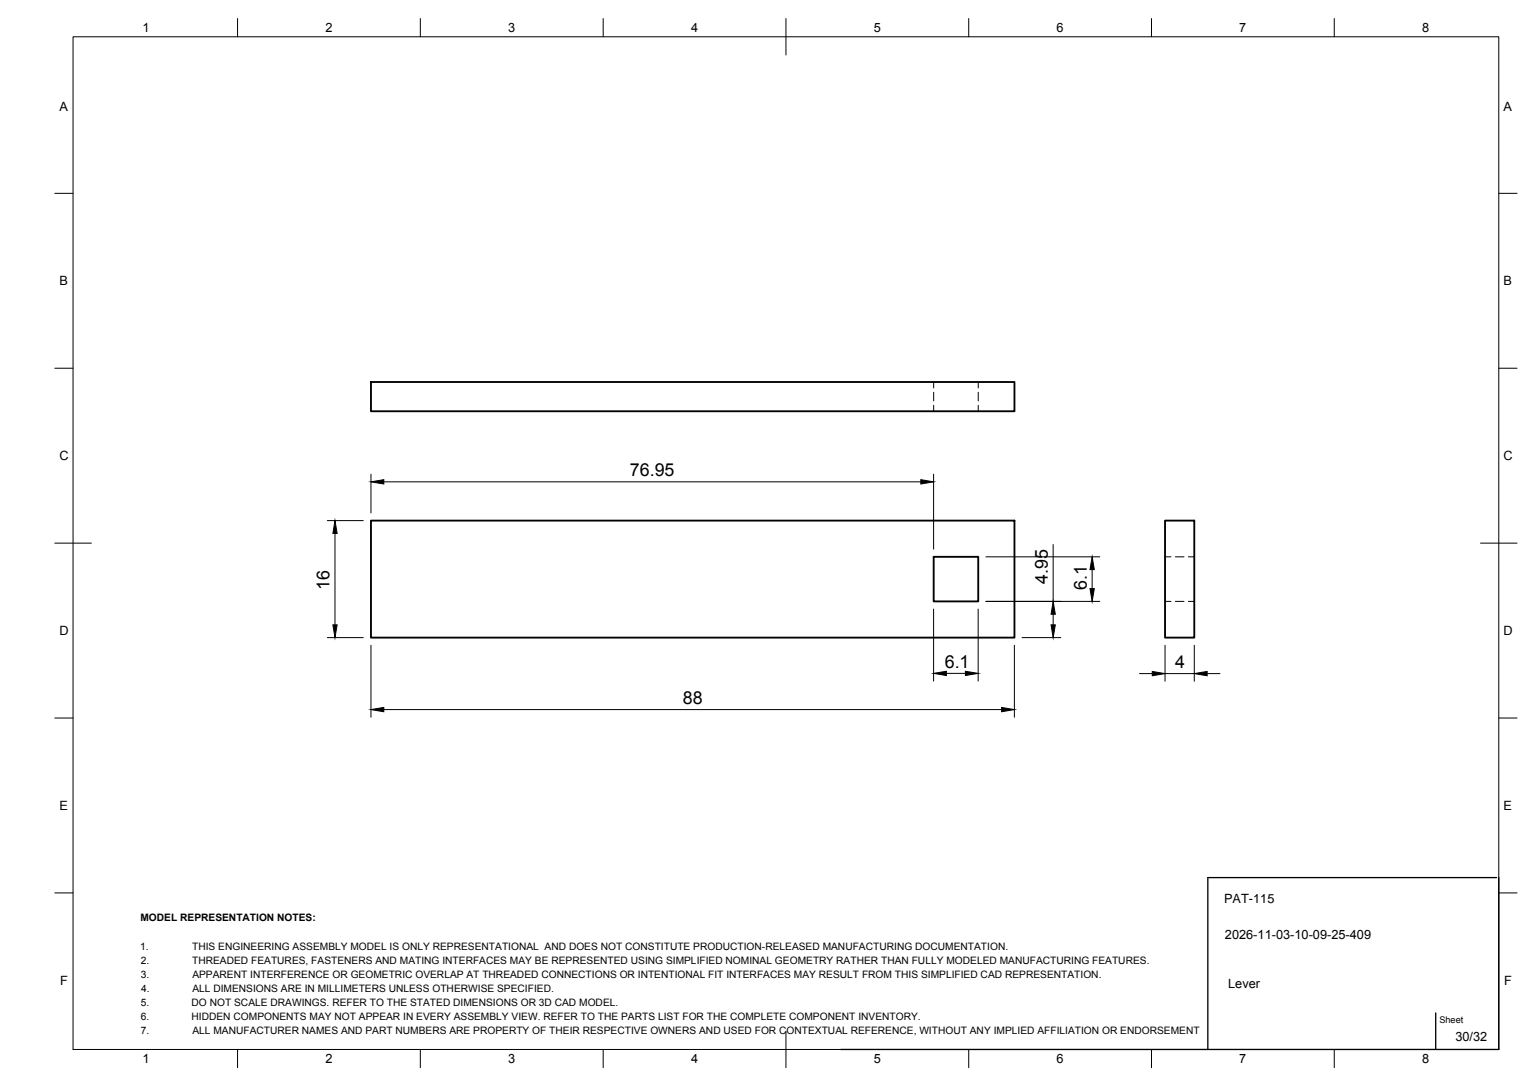
ISO-10303-21;
HEADER;
/* Generated by software containing ST-Developer
 * from STEP Tools, Inc. (www.steptools.com) 
 */

FILE_DESCRIPTION(
/* description */ ('Union bypass pipe loop'),
/* implementation_level */ '2;1');

FILE_NAME(
/* name */ 'Lever.step',
/* time_stamp */ '2026-10-27T21:00:29-07:00',
/* author */ (''),
/* organization */ (''),
/* preprocessor_version */ 'ST-DEVELOPER v20.2',
/* originating_system */ 'Autodesk Translation Framework v15.17.0.0',
/* authorisation */ '');

FILE_SCHEMA (('AUTOMOTIVE_DESIGN { 1 0 10303 214 3 1 1 }'));
ENDSEC;

DATA;
#10=MECHANICAL_DESIGN_GEOMETRIC_PRESENTATION_REPRESENTATION('',(#473),#10095);
#409=SHAPE_REPRESENTATION_RELATIONSHIP('SRR','None',#10279,#441);
#441=ADVANCED_BREP_SHAPE_REPRESENTATION('',(#502),#10091);
#473=STYLED_ITEM('',(#10514),#502);
#502=MANIFOLD_SOLID_BREP('Body1',#5547);
#630=FACE_BOUND('',#1591,.T.);
#631=FACE_BOUND('',#1593,.T.);
#806=PLANE('',#6561);
#807=PLANE('',#6562);
#808=PLANE('',#6563);
#809=PLANE('',#6564);
#810=PLANE('',#6565);
#811=PLANE('',#6566);
#812=PLANE('',#6567);
#813=PLANE('',#6568);
#814=PLANE('',#6569);
#815=PLANE('',#6570);
#1131=FACE_OUTER_BOUND('',#1582,.T.);
#1132=FACE_OUTER_BOUND('',#1583,.T.);
#1133=FACE_OUTER_BOUND('',#1584,.T.);
#1134=FACE_OUTER_BOUND('',#1585,.T.);
#1135=FACE_OUTER_BOUND('',#1586,.T.);
#1136=FACE_OUTER_BOUND('',#1587,.T.);
#1137=FACE_OUTER_BOUND('',#1588,.T.);
#1138=FACE_OUTER_BOUND('',#1589,.T.);
#1139=FACE_OUTER_BOUND('',#1590,.T.);
#1140=FACE_OUTER_BOUND('',#1592,.T.);
#1582=EDGE_LOOP('',(#4936,#4937,#4938,#4939));
#1583=EDGE_LOOP('',(#4940,#4941,#4942,#4943));
#1584=EDGE_LOOP('',(#4944,#4945,#4946,#4947));
#1585=EDGE_LOOP('',(#4948,#4949,#4950,#4951));
#1586=EDGE_LOOP('',(#4952,#4953,#4954,#4955));
#1587=EDGE_LOOP('',(#4956,#4957,#4958,#4959));
#1588=EDGE_LOOP('',(#4960,#4961,#4962,#4963));
#1589=EDGE_LOOP('',(#4964,#4965,#4966,#4967));
#1590=EDGE_LOOP('',(#4968,#4969,#4970,#4971));
#1591=EDGE_LOOP('',(#4972,#4973,#4974,#4975));
#1592=EDGE_LOOP('',(#4976,#4977,#4978,#4979));
#1593=EDGE_LOOP('',(#4980,#4981,#4982,#4983));
#1938=LINE('',#9859,#2314);
#1939=LINE('',#9861,#2315);
#1940=LINE('',#9863,#2316);
#1941=LINE('',#9864,#2317);
#1942=LINE('',#9867,#2318);
#1943=LINE('',#9869,#2319);
#1944=LINE('',#9870,#2320);
#1945=LINE('',#9873,#2321);
#1946=LINE('',#9875,#2322);
#1947=LINE('',#9876,#2323);
#1948=LINE('',#9878,#2324);
#1949=LINE('',#9879,#2325);
#1950=LINE('',#9883,#2326);
#1951=LINE('',#9885,#2327);
#1952=LINE('',#9887,#2328);
#1953=LINE('',#9888,#2329);
#1954=LINE('',#9891,#2330);
#1955=LINE('',#9893,#2331);
#1956=LINE('',#9894,#2332);
#1957=LINE('',#9897,#2333);
#1958=LINE('',#9899,#2334);
#1959=LINE('',#9900,#2335);
#1960=LINE('',#9902,#2336);
#1961=LINE('',#9903,#2337);
#2314=VECTOR('',#8248,1.);
#2315=VECTOR('',#8249,1.);
#2316=VECTOR('',#8250,1.);
#2317=VECTOR('',#8251,1.);
#2318=VECTOR('',#8254,1.);
#2319=VECTOR('',#8255,1.);
#2320=VECTOR('',#8256,1.);
#2321=VECTOR('',#8259,1.);
#2322=VECTOR('',#8260,1.);
#2323=VECTOR('',#8261,1.);
#2324=VECTOR('',#8264,1.);
#2325=VECTOR('',#8265,1.);
#2326=VECTOR('',#8268,1.);
#2327=VECTOR('',#8269,1.);
#2328=VECTOR('',#8270,1.);
#2329=VECTOR('',#8271,1.);
#2330=VECTOR('',#8274,1.);
#2331=VECTOR('',#8275,1.);
#2332=VECTOR('',#8276,1.);
#2333=VECTOR('',#8279,1.);
#2334=VECTOR('',#8280,1.);
#2335=VECTOR('',#8281,1.);
#2336=VECTOR('',#8284,1.);
#2337=VECTOR('',#8285,1.);
#3020=VERTEX_POINT('',#9857);
#3021=VERTEX_POINT('',#9858);
#3022=VERTEX_POINT('',#9860);
#3023=VERTEX_POINT('',#9862);
#3024=VERTEX_POINT('',#9866);
#3025=VERTEX_POINT('',#9868);
#3026=VERTEX_POINT('',#9872);
#3027=VERTEX_POINT('',#9874);
#3028=VERTEX_POINT('',#9881);
#3029=VERTEX_POINT('',#9882);
#3030=VERTEX_POINT('',#9884);
#3031=VERTEX_POINT('',#9886);
#3032=VERTEX_POINT('',#9890);
#3033=VERTEX_POINT('',#9892);
#3034=VERTEX_POINT('',#9896);
#3035=VERTEX_POINT('',#9898);
#3666=EDGE_CURVE('',#3020,#3021,#1938,.T.);
#3667=EDGE_CURVE('',#3022,#3020,#1939,.T.);
#3668=EDGE_CURVE('',#3023,#3022,#1940,.T.);
#3669=EDGE_CURVE('',#3023,#3021,#1941,.T.);
#3670=EDGE_CURVE('',#3021,#3024,#1942,.T.);
#3671=EDGE_CURVE('',#3025,#3023,#1943,.T.);
#3672=EDGE_CURVE('',#3025,#3024,#1944,.T.);
#3673=EDGE_CURVE('',#3024,#3026,#1945,.T.);
#3674=EDGE_CURVE('',#3027,#3025,#1946,.T.);
#3675=EDGE_CURVE('',#3027,#3026,#1947,.T.);
#3676=EDGE_CURVE('',#3026,#3020,#1948,.T.);
#3677=EDGE_CURVE('',#3022,#3027,#1949,.T.);
#3678=EDGE_CURVE('',#3028,#3029,#1950,.T.);
#3679=EDGE_CURVE('',#3029,#3030,#1951,.T.);
#3680=EDGE_CURVE('',#3031,#3030,#1952,.T.);
#3681=EDGE_CURVE('',#3028,#3031,#1953,.T.);
#3682=EDGE_CURVE('',#3032,#3028,#1954,.T.);
#3683=EDGE_CURVE('',#3033,#3031,#1955,.T.);
#3684=EDGE_CURVE('',#3032,#3033,#1956,.T.);
#3685=EDGE_CURVE('',#3034,#3032,#1957,.T.);
#3686=EDGE_CURVE('',#3035,#3033,#1958,.T.);
#3687=EDGE_CURVE('',#3034,#3035,#1959,.T.);
#3688=EDGE_CURVE('',#3029,#3034,#1960,.T.);
#3689=EDGE_CURVE('',#3030,#3035,#1961,.T.);
#4936=ORIENTED_EDGE('',*,*,#3666,.F.);
#4937=ORIENTED_EDGE('',*,*,#3667,.F.);
#4938=ORIENTED_EDGE('',*,*,#3668,.F.);
#4939=ORIENTED_EDGE('',*,*,#3669,.T.);
#4940=ORIENTED_EDGE('',*,*,#3670,.F.);
#4941=ORIENTED_EDGE('',*,*,#3669,.F.);
#4942=ORIENTED_EDGE('',*,*,#3671,.F.);
#4943=ORIENTED_EDGE('',*,*,#3672,.T.);
#4944=ORIENTED_EDGE('',*,*,#3673,.F.);
#4945=ORIENTED_EDGE('',*,*,#3672,.F.);
#4946=ORIENTED_EDGE('',*,*,#3674,.F.);
#4947=ORIENTED_EDGE('',*,*,#3675,.T.);
#4948=ORIENTED_EDGE('',*,*,#3676,.F.);
#4949=ORIENTED_EDGE('',*,*,#3675,.F.);
#4950=ORIENTED_EDGE('',*,*,#3677,.F.);
#4951=ORIENTED_EDGE('',*,*,#3667,.T.);
#4952=ORIENTED_EDGE('',*,*,#3678,.T.);
#4953=ORIENTED_EDGE('',*,*,#3679,.T.);
#4954=ORIENTED_EDGE('',*,*,#3680,.F.);
#4955=ORIENTED_EDGE('',*,*,#3681,.F.);
#4956=ORIENTED_EDGE('',*,*,#3682,.T.);
#4957=ORIENTED_EDGE('',*,*,#3681,.T.);
#4958=ORIENTED_EDGE('',*,*,#3683,.F.);
#4959=ORIENTED_EDGE('',*,*,#3684,.F.);
#4960=ORIENTED_EDGE('',*,*,#3685,.T.);
#4961=ORIENTED_EDGE('',*,*,#3684,.T.);
#4962=ORIENTED_EDGE('',*,*,#3686,.F.);
#4963=ORIENTED_EDGE('',*,*,#3687,.F.);
#4964=ORIENTED_EDGE('',*,*,#3688,.T.);
#4965=ORIENTED_EDGE('',*,*,#3687,.T.);
#4966=ORIENTED_EDGE('',*,*,#3689,.F.);
#4967=ORIENTED_EDGE('',*,*,#3679,.F.);
#4968=ORIENTED_EDGE('',*,*,#3689,.T.);
#4969=ORIENTED_EDGE('',*,*,#3686,.T.);
#4970=ORIENTED_EDGE('',*,*,#3683,.T.);
#4971=ORIENTED_EDGE('',*,*,#3680,.T.);
#4972=ORIENTED_EDGE('',*,*,#3673,.T.);
#4973=ORIENTED_EDGE('',*,*,#3676,.T.);
#4974=ORIENTED_EDGE('',*,*,#3666,.T.);
#4975=ORIENTED_EDGE('',*,*,#3670,.T.);
#4976=ORIENTED_EDGE('',*,*,#3688,.F.);
#4977=ORIENTED_EDGE('',*,*,#3678,.F.);
#4978=ORIENTED_EDGE('',*,*,#3682,.F.);
#4979=ORIENTED_EDGE('',*,*,#3685,.F.);
#4980=ORIENTED_EDGE('',*,*,#3674,.T.);
#4981=ORIENTED_EDGE('',*,*,#3671,.T.);
#4982=ORIENTED_EDGE('',*,*,#3668,.T.);
#4983=ORIENTED_EDGE('',*,*,#3677,.T.);
#5480=ADVANCED_FACE('',(#1131),#806,.F.);
#5481=ADVANCED_FACE('',(#1132),#807,.F.);
#5482=ADVANCED_FACE('',(#1133),#808,.F.);
#5483=ADVANCED_FACE('',(#1134),#809,.F.);
#5484=ADVANCED_FACE('',(#1135),#810,.T.);
#5485=ADVANCED_FACE('',(#1136),#811,.T.);
#5486=ADVANCED_FACE('',(#1137),#812,.T.);
#5487=ADVANCED_FACE('',(#1138),#813,.T.);
#5488=ADVANCED_FACE('',(#1139,#630),#814,.T.);
#5489=ADVANCED_FACE('',(#1140,#631),#815,.F.);
#5547=CLOSED_SHELL('',(#5480,#5481,#5482,#5483,#5484,#5485,#5486,#5487,
#5488,#5489));
#6560=AXIS2_PLACEMENT_3D('',#9855,#8244,#8245);
#6561=AXIS2_PLACEMENT_3D('',#9856,#8246,#8247);
#6562=AXIS2_PLACEMENT_3D('',#9865,#8252,#8253);
#6563=AXIS2_PLACEMENT_3D('',#9871,#8257,#8258);
#6564=AXIS2_PLACEMENT_3D('',#9877,#8262,#8263);
#6565=AXIS2_PLACEMENT_3D('',#9880,#8266,#8267);
#6566=AXIS2_PLACEMENT_3D('',#9889,#8272,#8273);
#6567=AXIS2_PLACEMENT_3D('',#9895,#8277,#8278);
#6568=AXIS2_PLACEMENT_3D('',#9901,#8282,#8283);
#6569=AXIS2_PLACEMENT_3D('',#9904,#8286,#8287);
#6570=AXIS2_PLACEMENT_3D('',#9905,#8288,#8289);
#8244=DIRECTION('axis',(0.,0.,1.));
#8245=DIRECTION('refdir',(1.,0.,0.));
#8246=DIRECTION('center_axis',(0.,-1.,0.));
#8247=DIRECTION('ref_axis',(1.,0.,0.));
#8248=DIRECTION('',(-1.,0.,0.));
#8249=DIRECTION('',(0.,0.,1.));
#8250=DIRECTION('',(1.,0.,0.));
#8251=DIRECTION('',(0.,0.,1.));
#8252=DIRECTION('center_axis',(-1.,0.,0.));
#8253=DIRECTION('ref_axis',(0.,-1.,0.));
#8254=DIRECTION('',(0.,1.,0.));
#8255=DIRECTION('',(0.,-1.,0.));
#8256=DIRECTION('',(0.,0.,1.));
#8257=DIRECTION('center_axis',(0.,1.,0.));
#8258=DIRECTION('ref_axis',(-1.,0.,0.));
#8259=DIRECTION('',(1.,0.,0.));
#8260=DIRECTION('',(-1.,0.,0.));
#8261=DIRECTION('',(0.,0.,1.));
#8262=DIRECTION('center_axis',(1.,0.,0.));
#8263=DIRECTION('ref_axis',(0.,1.,0.));
#8264=DIRECTION('',(0.,-1.,0.));
#8265=DIRECTION('',(0.,1.,0.));
#8266=DIRECTION('center_axis',(0.,1.,0.));
#8267=DIRECTION('ref_axis',(-1.,0.,0.));
#8268=DIRECTION('',(-1.,0.,0.));
#8269=DIRECTION('',(0.,0.,1.));
#8270=DIRECTION('',(-1.,0.,0.));
#8271=DIRECTION('',(0.,0.,1.));
#8272=DIRECTION('center_axis',(1.,0.,0.));
#8273=DIRECTION('ref_axis',(0.,1.,0.));
#8274=DIRECTION('',(0.,1.,0.));
#8275=DIRECTION('',(0.,1.,0.));
#8276=DIRECTION('',(0.,0.,1.));
#8277=DIRECTION('center_axis',(0.,-1.,0.));
#8278=DIRECTION('ref_axis',(1.,0.,0.));
#8279=DIRECTION('',(1.,0.,0.));
#8280=DIRECTION('',(1.,0.,0.));
#8281=DIRECTION('',(0.,0.,1.));
#8282=DIRECTION('center_axis',(-1.,0.,0.));
#8283=DIRECTION('ref_axis',(0.,-1.,0.));
#8284=DIRECTION('',(0.,-1.,0.));
#8285=DIRECTION('',(0.,-1.,0.));
#8286=DIRECTION('center_axis',(0.,0.,1.));
#8287=DIRECTION('ref_axis',(1.,0.,0.));
#8288=DIRECTION('center_axis',(0.,0.,1.));
#8289=DIRECTION('ref_axis',(1.,0.,0.));
#9855=CARTESIAN_POINT('',(0.,0.,0.));
#9856=CARTESIAN_POINT('Origin',(-0.305,-0.305,8.9));
#9857=CARTESIAN_POINT('',(0.305,-0.305,9.4));
#9858=CARTESIAN_POINT('',(-0.305,-0.305,9.4));
#9859=CARTESIAN_POINT('',(1.6475,-0.305,9.4));
#9860=CARTESIAN_POINT('',(0.305,-0.305,9.));
#9861=CARTESIAN_POINT('',(0.305,-0.305,8.9));
#9862=CARTESIAN_POINT('',(-0.305,-0.305,9.));
#9863=CARTESIAN_POINT('',(1.6475,-0.305,9.));
#9864=CARTESIAN_POINT('',(-0.305,-0.305,8.9));
#9865=CARTESIAN_POINT('Origin',(-0.305,0.305,8.9));
#9866=CARTESIAN_POINT('',(-0.305,0.305,9.4));
#9867=CARTESIAN_POINT('',(-0.305,0.1525,9.4));
#9868=CARTESIAN_POINT('',(-0.305,0.305,9.));
#9869=CARTESIAN_POINT('',(-0.305,0.1525,9.));
#9870=CARTESIAN_POINT('',(-0.305,0.305,8.9));
#9871=CARTESIAN_POINT('Origin',(0.305,0.305,8.9));
#9872=CARTESIAN_POINT('',(0.305,0.305,9.4));
#9873=CARTESIAN_POINT('',(1.9525,0.305,9.4));
#9874=CARTESIAN_POINT('',(0.305,0.305,9.));
#9875=CARTESIAN_POINT('',(1.9525,0.305,9.));
#9876=CARTESIAN_POINT('',(0.305,0.305,8.9));
#9877=CARTESIAN_POINT('Origin',(0.305,-0.305,8.9));
#9878=CARTESIAN_POINT('',(0.305,-0.1525,9.4));
#9879=CARTESIAN_POINT('',(0.305,-0.1525,9.));
#9880=CARTESIAN_POINT('Origin',(8.,0.8,9.));
#9881=CARTESIAN_POINT('',(8.,0.8,9.));
#9882=CARTESIAN_POINT('',(-0.8,0.8,9.));
#9883=CARTESIAN_POINT('',(8.,0.8,9.));
#9884=CARTESIAN_POINT('',(-0.8,0.8,9.4));
#9885=CARTESIAN_POINT('',(-0.8,0.8,9.));
#9886=CARTESIAN_POINT('',(8.,0.8,9.4));
#9887=CARTESIAN_POINT('',(8.,0.8,9.4));
#9888=CARTESIAN_POINT('',(8.,0.8,9.));
#9889=CARTESIAN_POINT('Origin',(8.,-0.8,9.));
#9890=CARTESIAN_POINT('',(8.,-0.8,9.));
#9891=CARTESIAN_POINT('',(8.,-0.8,9.));
#9892=CARTESIAN_POINT('',(8.,-0.8,9.4));
#9893=CARTESIAN_POINT('',(8.,-0.8,9.4));
#9894=CARTESIAN_POINT('',(8.,-0.8,9.));
#9895=CARTESIAN_POINT('Origin',(-0.8,-0.8,9.));
#9896=CARTESIAN_POINT('',(-0.8,-0.8,9.));
#9897=CARTESIAN_POINT('',(-0.8,-0.8,9.));
#9898=CARTESIAN_POINT('',(-0.8,-0.8,9.4));
#9899=CARTESIAN_POINT('',(-0.8,-0.8,9.4));
#9900=CARTESIAN_POINT('',(-0.8,-0.8,9.));
#9901=CARTESIAN_POINT('Origin',(-0.8,0.8,9.));
#9902=CARTESIAN_POINT('',(-0.8,0.8,9.));
#9903=CARTESIAN_POINT('',(-0.8,0.8,9.4));
#9904=CARTESIAN_POINT('Origin',(3.6,0.,9.4));
#9905=CARTESIAN_POINT('Origin',(3.6,0.,9.));
#10054=UNCERTAINTY_MEASURE_WITH_UNIT(LENGTH_MEASURE(0.001),#10096,
'DISTANCE_ACCURACY_VALUE',
'Maximum model space distance between geometric entities at asserted c
onnectivities');
#10058=UNCERTAINTY_MEASURE_WITH_UNIT(LENGTH_MEASURE(0.001),#10096,
'DISTANCE_ACCURACY_VALUE',
'Maximum model space distance between geometric entities at asserted c
onnectivities');
#10091=(
GEOMETRIC_REPRESENTATION_CONTEXT(3)
GLOBAL_UNCERTAINTY_ASSIGNED_CONTEXT((#10054))
GLOBAL_UNIT_ASSIGNED_CONTEXT((#10096,#10098,#10099))
REPRESENTATION_CONTEXT('','3D')
);
#10095=(
GEOMETRIC_REPRESENTATION_CONTEXT(3)
GLOBAL_UNCERTAINTY_ASSIGNED_CONTEXT((#10058))
GLOBAL_UNIT_ASSIGNED_CONTEXT((#10096,#10098,#10099))
REPRESENTATION_CONTEXT('','3D')
);
#10096=(
LENGTH_UNIT()
NAMED_UNIT(*)
SI_UNIT(.CENTI.,.METRE.)
);
#10098=(
NAMED_UNIT(*)
PLANE_ANGLE_UNIT()
SI_UNIT($,.RADIAN.)
);
#10099=(
NAMED_UNIT(*)
SI_UNIT($,.STERADIAN.)
SOLID_ANGLE_UNIT()
);
#10132=SHAPE_DEFINITION_REPRESENTATION(#10235,#10279);
#10235=PRODUCT_DEFINITION_SHAPE('',$,#10316);
#10279=SHAPE_REPRESENTATION('',(#6560),#10091);
#10283=PRODUCT_DEFINITION_CONTEXT('part definition',#10393,'design');
#10316=PRODUCT_DEFINITION('Lever','Lever',#10352,#10283);
#10352=PRODUCT_DEFINITION_FORMATION('',$,#10427);
#10393=APPLICATION_CONTEXT(
'Core Data for Automotive Mechanical Design Process');
#10394=PRODUCT_CONTEXT('part definition',#10393,'mechanical');
#10427=PRODUCT('Lever','Lever','Lever',(#10394));
#10508=COLOUR_RGB('Off White',0.89,0.88,0.83);
#10509=FILL_AREA_STYLE_COLOUR('',#10508);
#10510=FILL_AREA_STYLE('',(#10509));
#10511=SURFACE_STYLE_FILL_AREA(#10510);
#10512=SURFACE_SIDE_STYLE('',(#10511));
#10513=SURFACE_STYLE_USAGE(.BOTH.,#10512);
#10514=PRESENTATION_STYLE_ASSIGNMENT((#10513));
ENDSEC;
END-ISO-10303-21;
